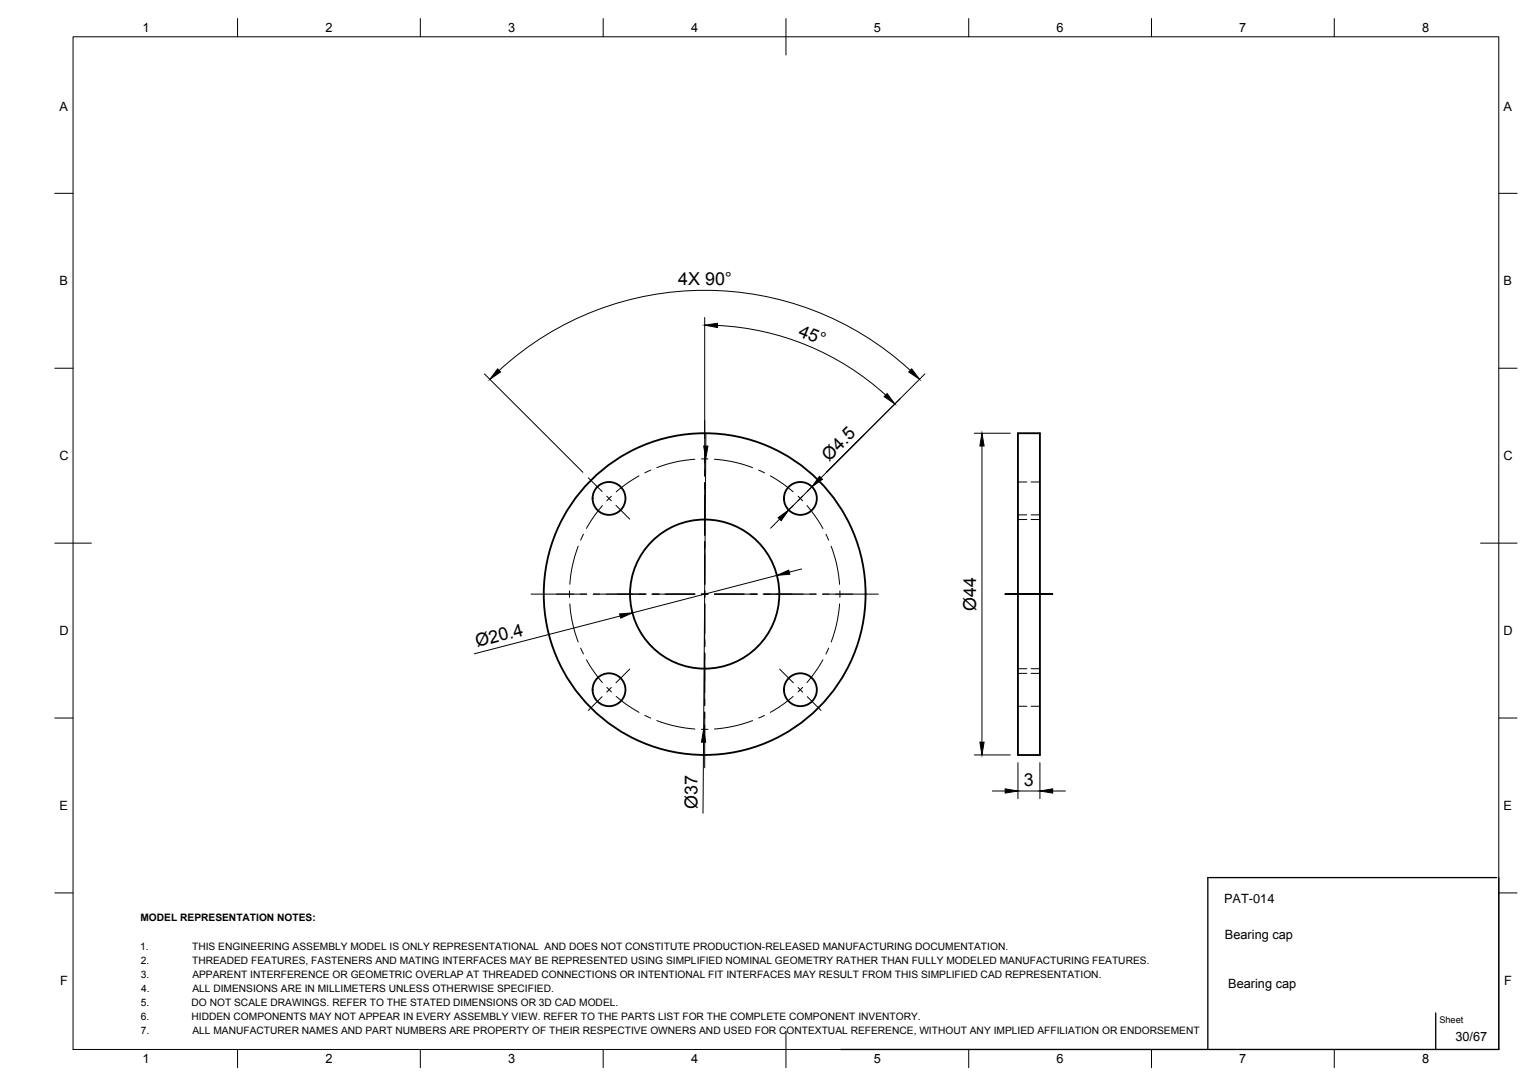
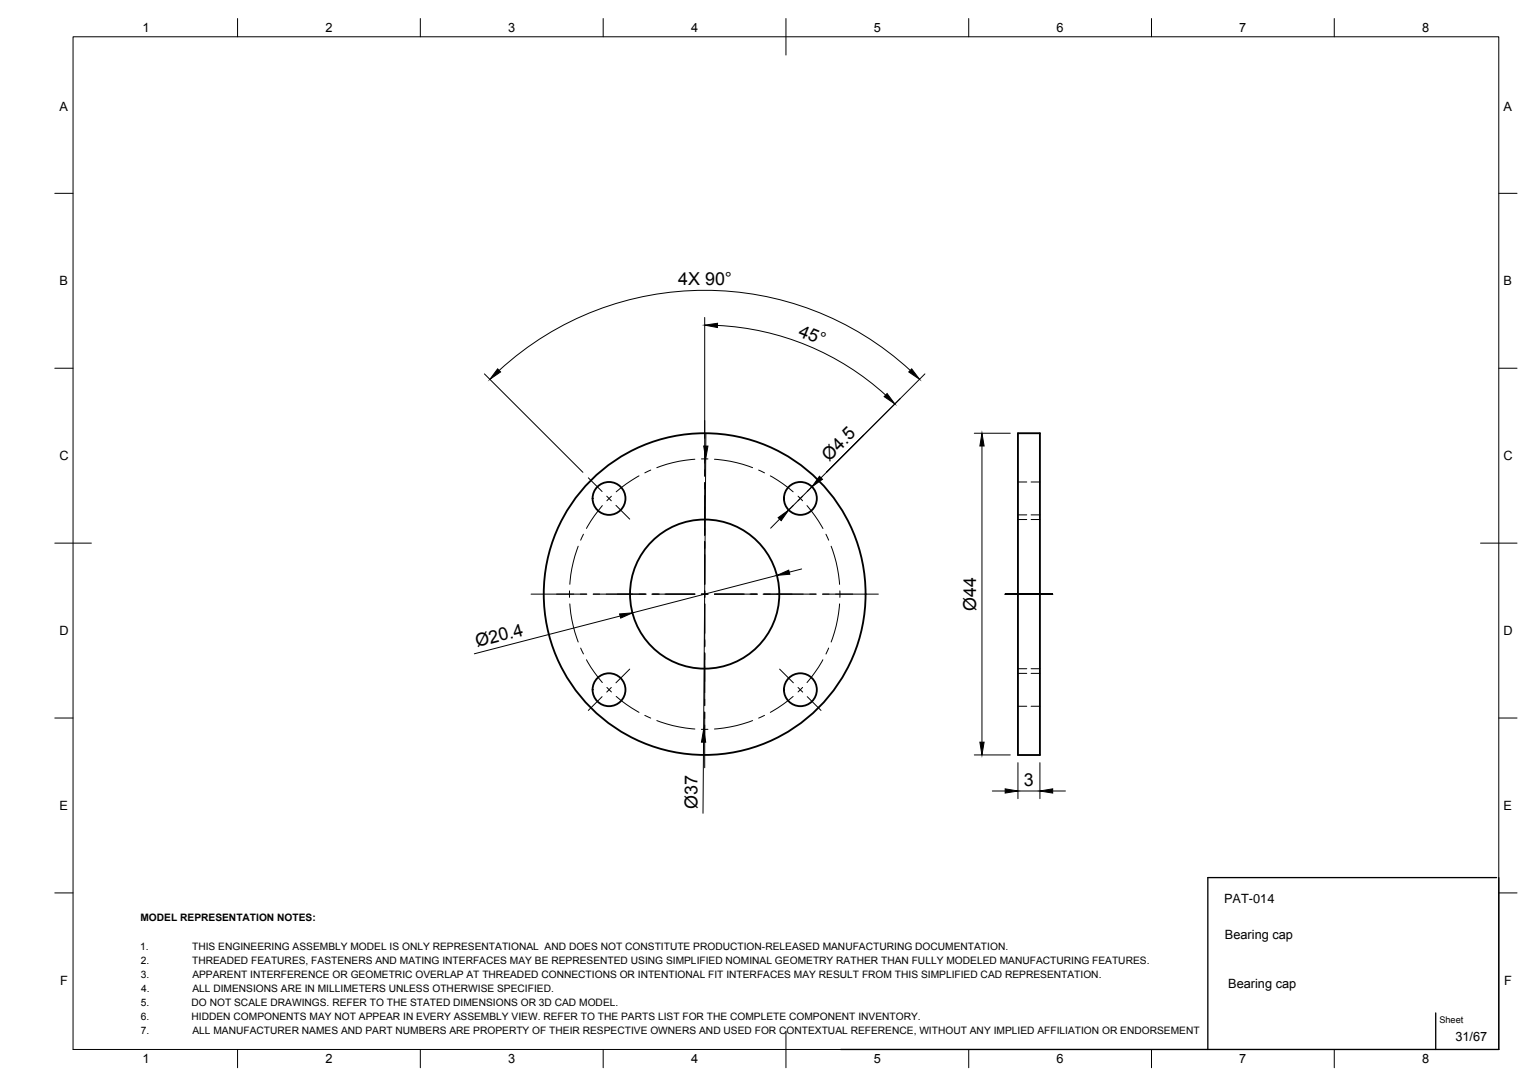
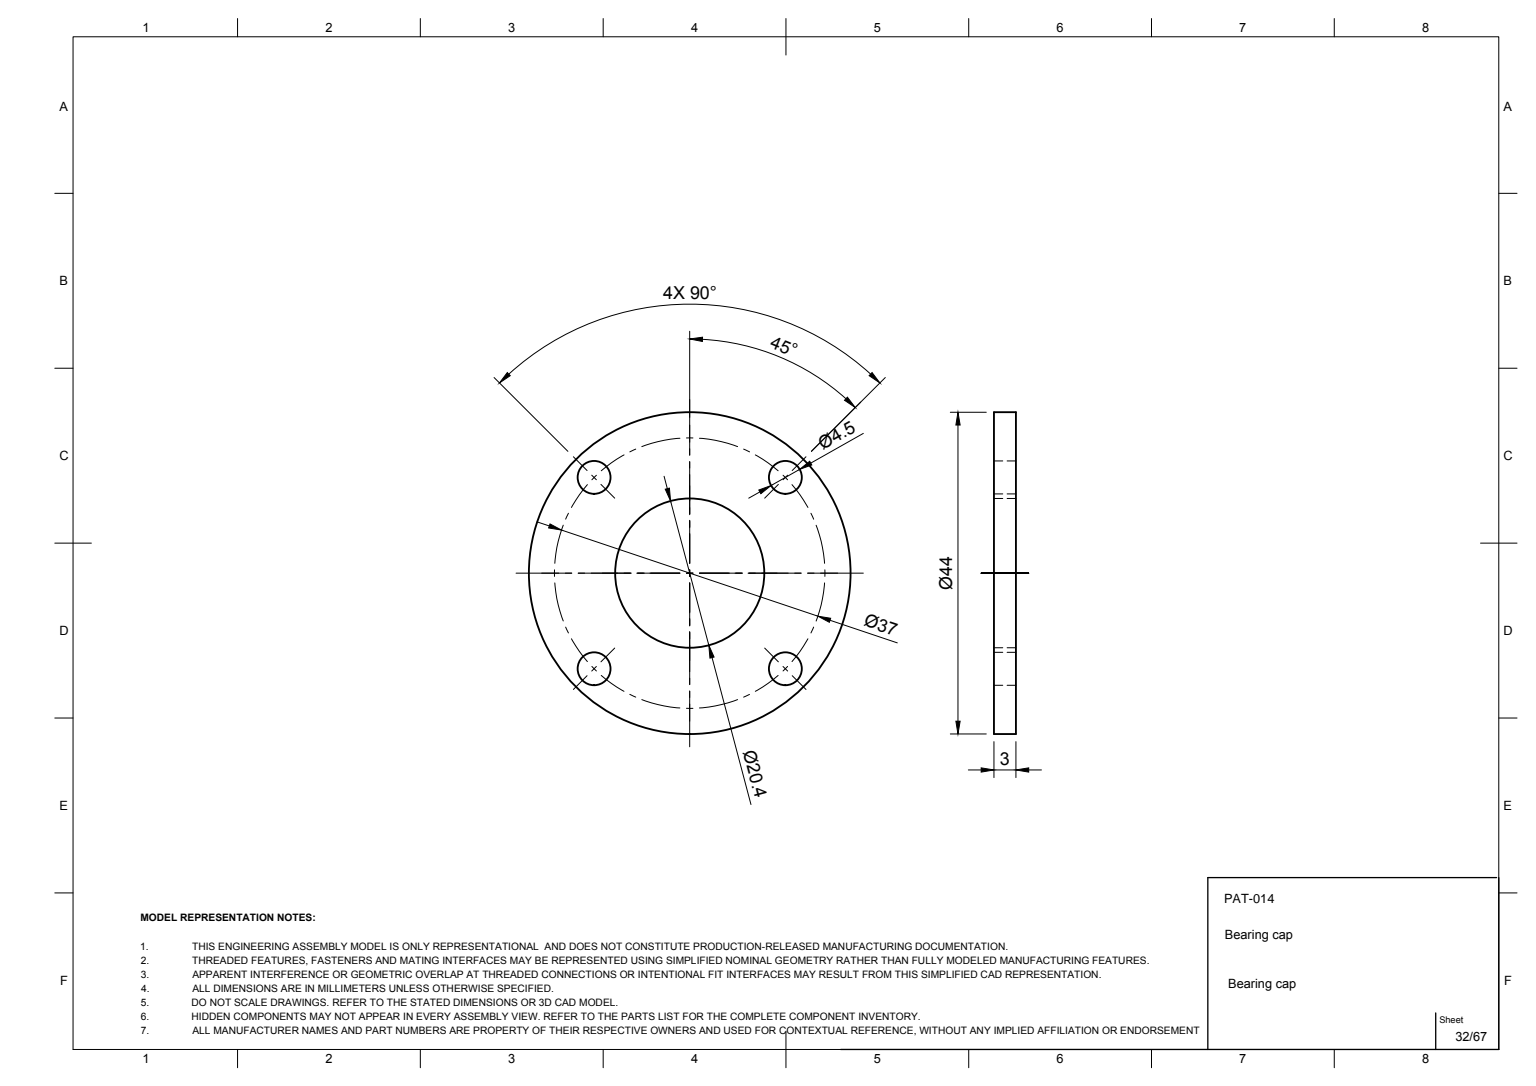
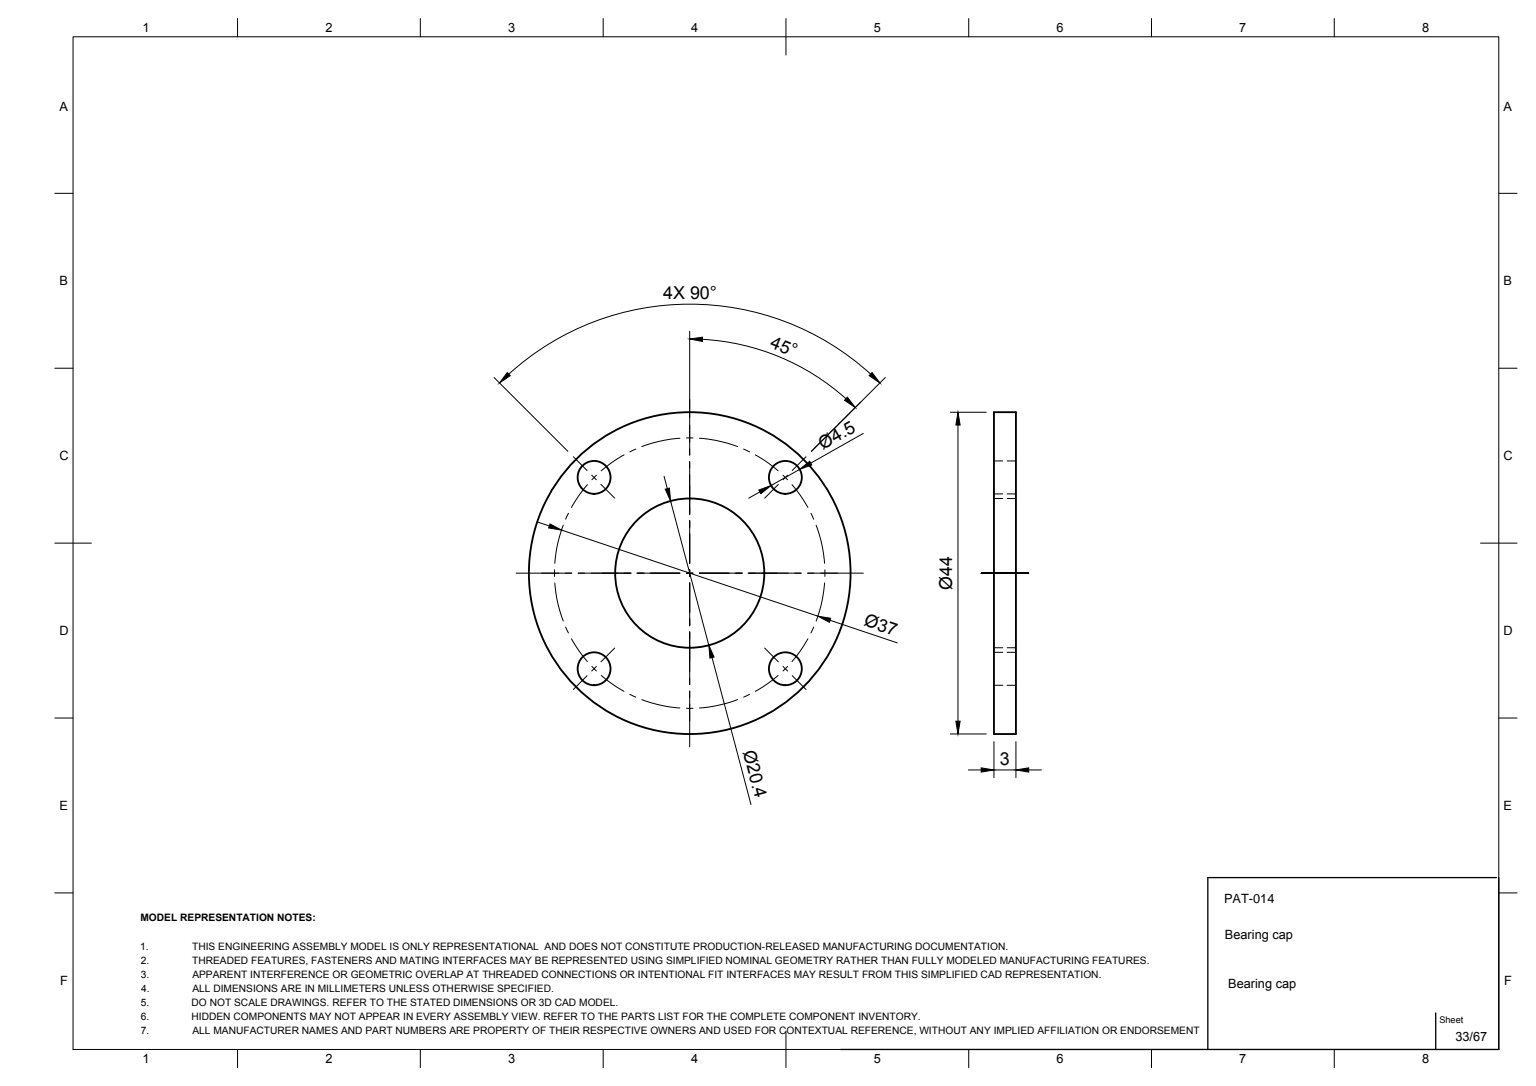
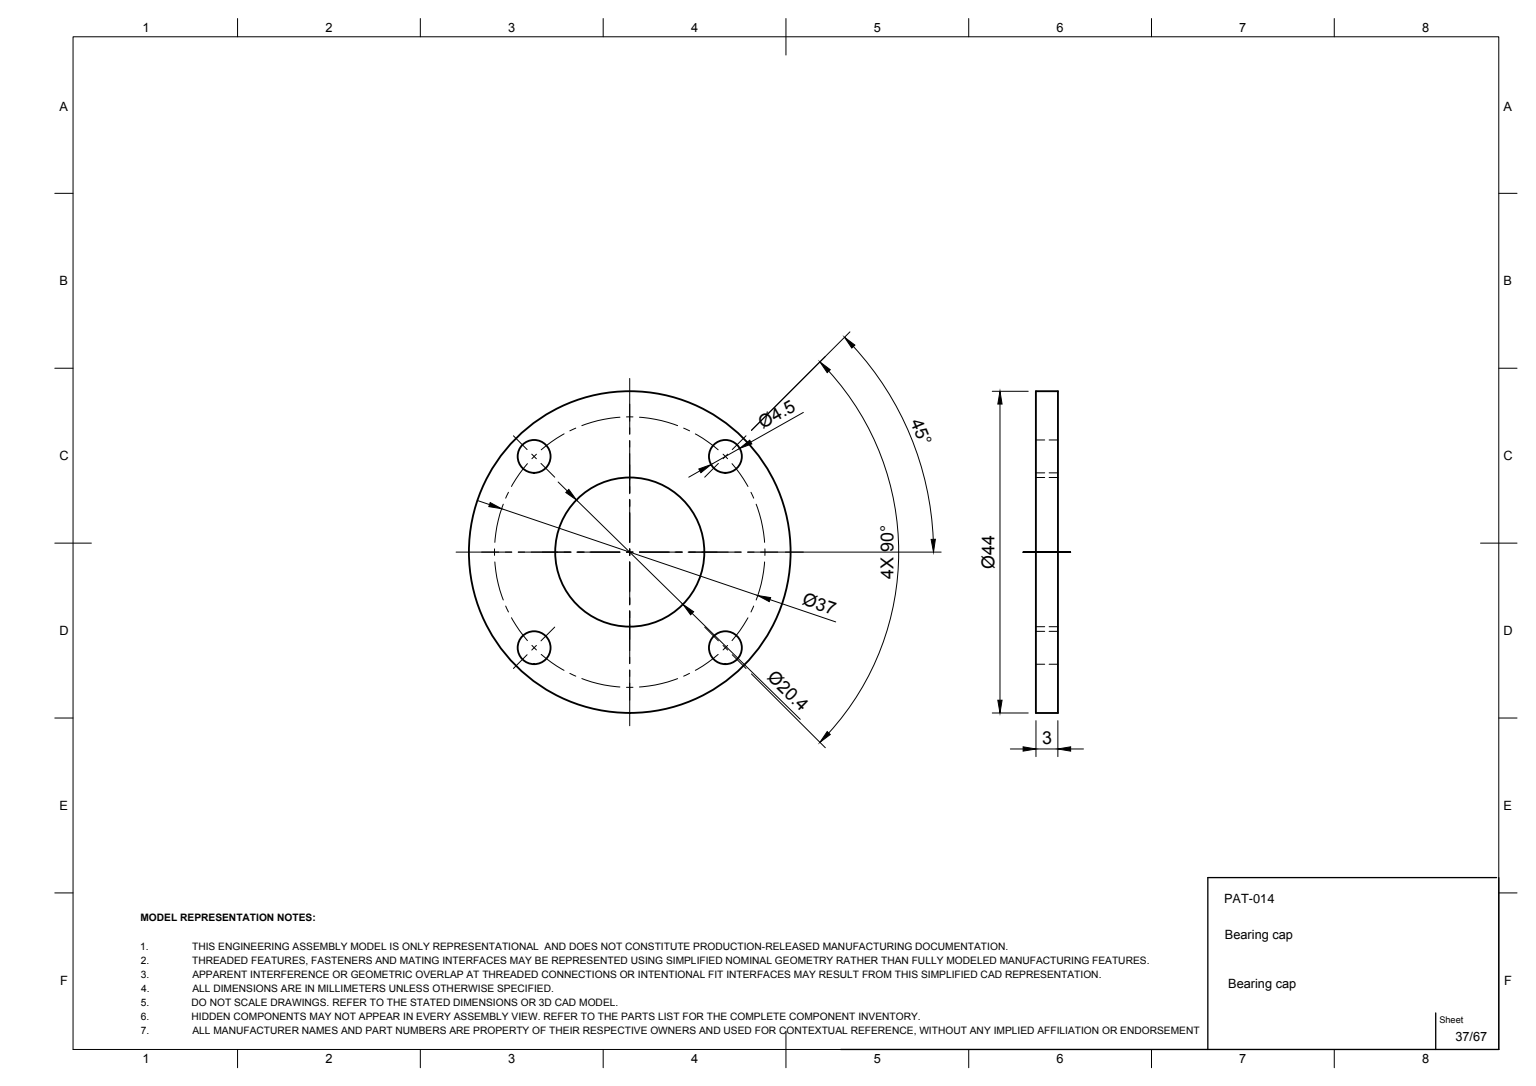
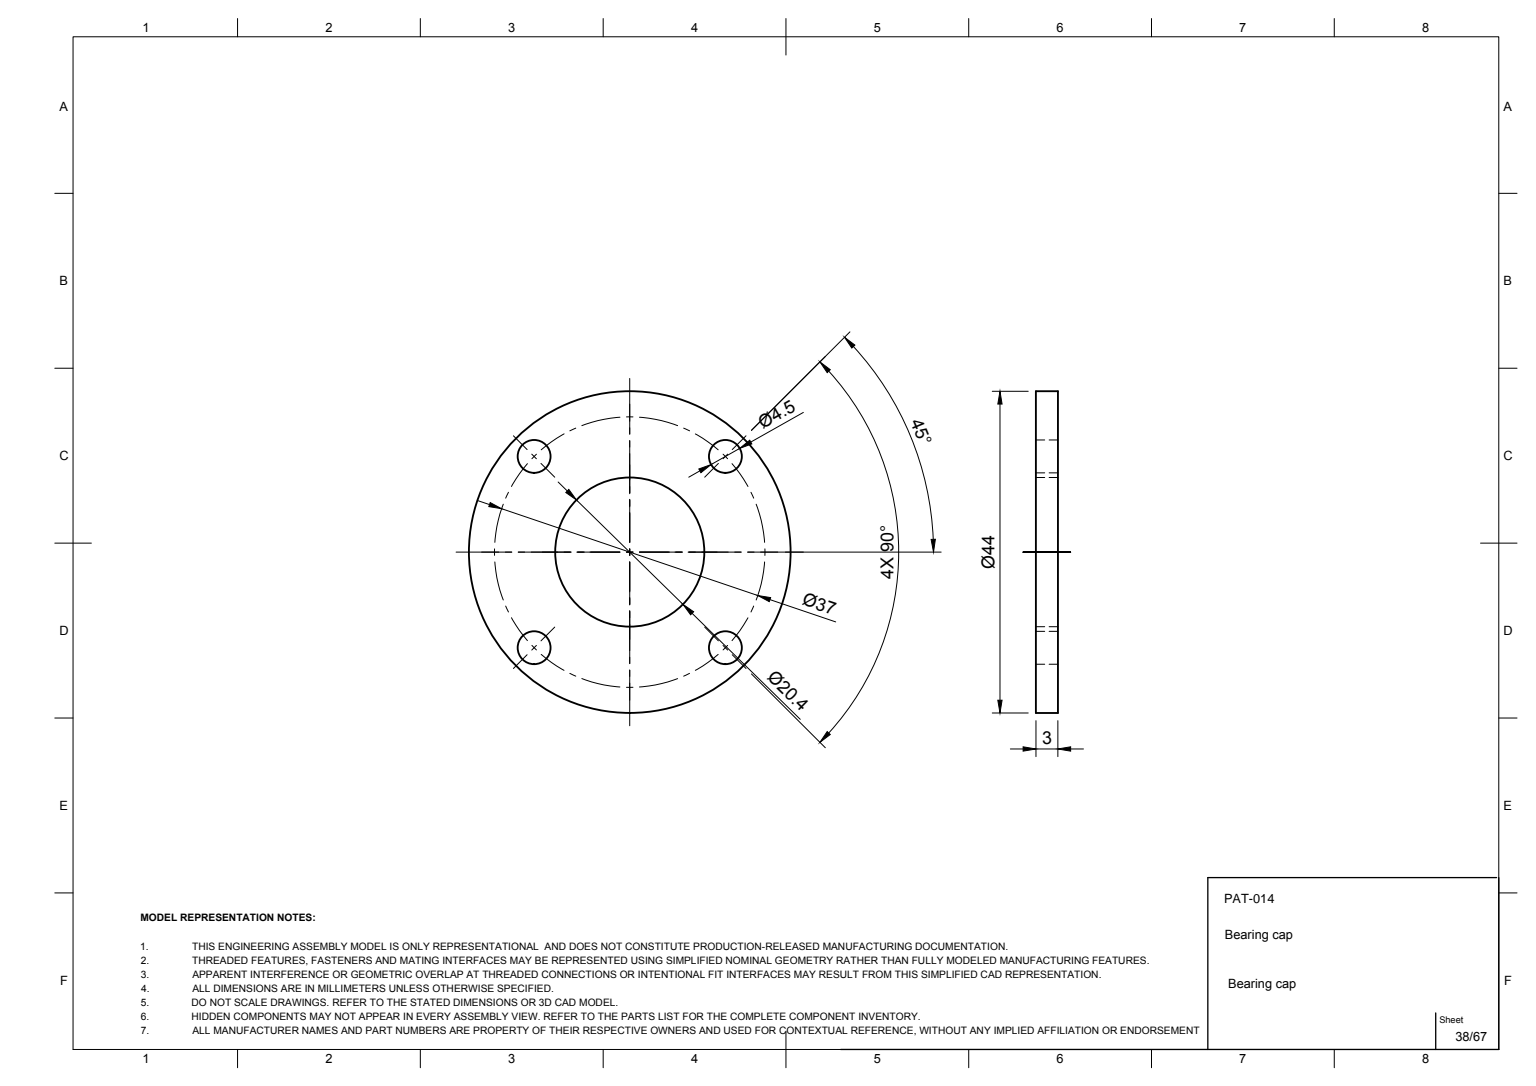
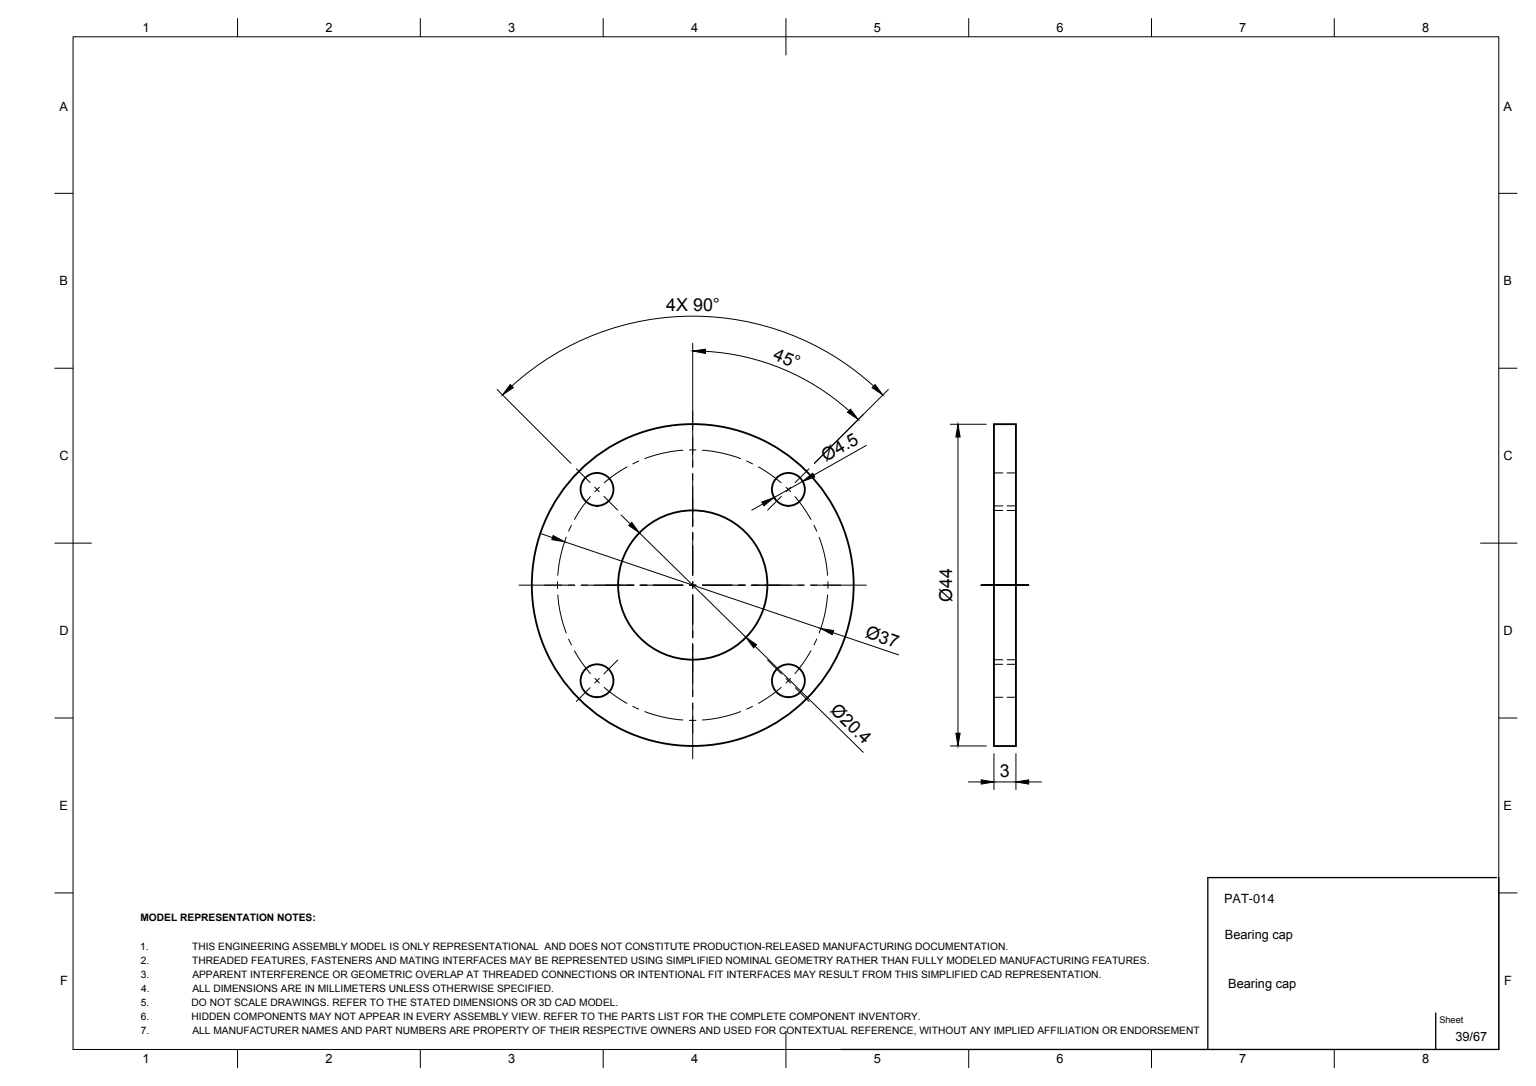
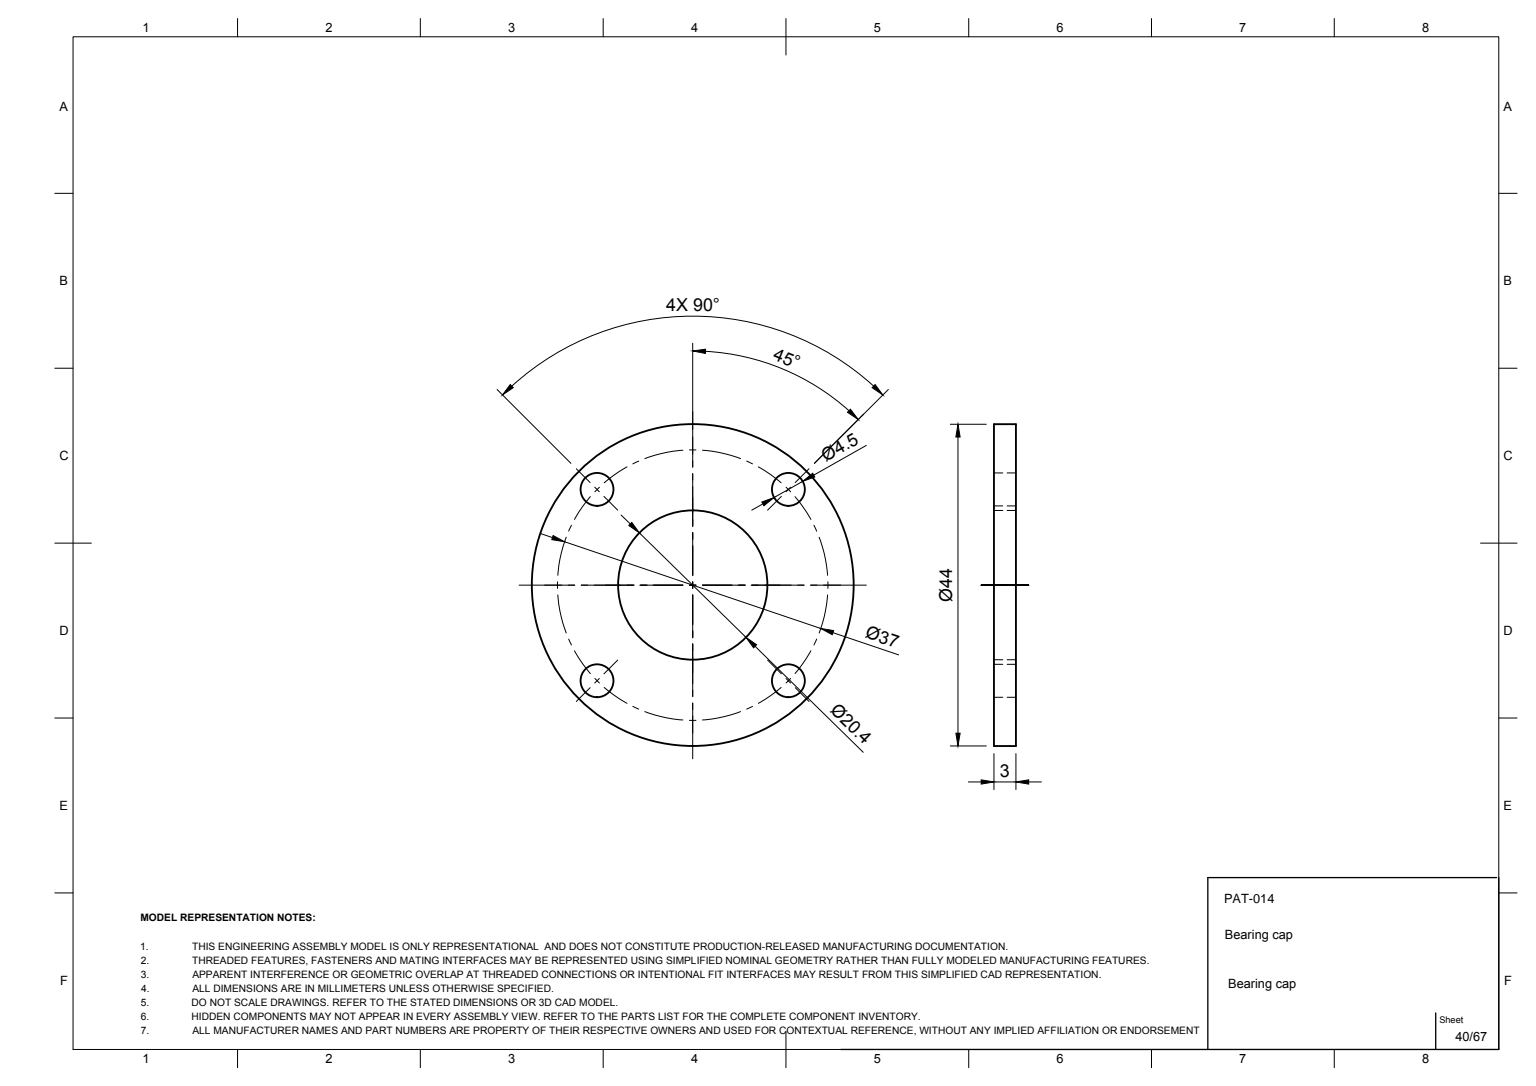
ISO-10303-21;
HEADER;
/* Generated by software containing ST-Developer
 * from STEP Tools, Inc. (www.steptools.com) 
 */

FILE_DESCRIPTION(
/* description */ ('Bin tilter linkage'),
/* implementation_level */ '2;1');

FILE_NAME(
/* name */ 'Bearing cap.step',
/* time_stamp */ '2026-10-28T03:26:24-07:00',
/* author */ (''),
/* organization */ (''),
/* preprocessor_version */ 'ST-DEVELOPER v20.2',
/* originating_system */ 'Autodesk Translation Framework v15.17.0.0',
/* authorisation */ '');

FILE_SCHEMA (('AUTOMOTIVE_DESIGN { 1 0 10303 214 3 1 1 }'));
ENDSEC;

DATA;
#10=MECHANICAL_DESIGN_GEOMETRIC_PRESENTATION_REPRESENTATION('',(#893),#23728);
#681=SHAPE_REPRESENTATION_RELATIONSHIP('SRR','None',#24146,#787);
#787=ADVANCED_BREP_SHAPE_REPRESENTATION('',(#1006),#23646);
#893=STYLED_ITEM('',(#24765),#1006);
#1006=MANIFOLD_SOLID_BREP('Body1',#12424);
#1254=FACE_BOUND('',#3106,.T.);
#1255=FACE_BOUND('',#3107,.T.);
#1256=FACE_BOUND('',#3108,.T.);
#1257=FACE_BOUND('',#3109,.T.);
#1258=FACE_BOUND('',#3110,.T.);
#1259=FACE_BOUND('',#3112,.T.);
#1260=FACE_BOUND('',#3113,.T.);
#1261=FACE_BOUND('',#3114,.T.);
#1262=FACE_BOUND('',#3115,.T.);
#1263=FACE_BOUND('',#3116,.T.);
#1621=PLANE('',#14262);
#1622=PLANE('',#14263);
#2155=FACE_OUTER_BOUND('',#3099,.T.);
#2156=FACE_OUTER_BOUND('',#3100,.T.);
#2157=FACE_OUTER_BOUND('',#3101,.T.);
#2158=FACE_OUTER_BOUND('',#3102,.T.);
#2159=FACE_OUTER_BOUND('',#3103,.T.);
#2160=FACE_OUTER_BOUND('',#3104,.T.);
#2161=FACE_OUTER_BOUND('',#3105,.T.);
#2162=FACE_OUTER_BOUND('',#3111,.T.);
#3099=EDGE_LOOP('',(#9457,#9458,#9459,#9460));
#3100=EDGE_LOOP('',(#9461,#9462,#9463,#9464));
#3101=EDGE_LOOP('',(#9465,#9466,#9467,#9468));
#3102=EDGE_LOOP('',(#9469,#9470,#9471,#9472));
#3103=EDGE_LOOP('',(#9473,#9474,#9475,#9476));
#3104=EDGE_LOOP('',(#9477,#9478,#9479,#9480));
#3105=EDGE_LOOP('',(#9481));
#3106=EDGE_LOOP('',(#9482));
#3107=EDGE_LOOP('',(#9483));
#3108=EDGE_LOOP('',(#9484));
#3109=EDGE_LOOP('',(#9485));
#3110=EDGE_LOOP('',(#9486));
#3111=EDGE_LOOP('',(#9487));
#3112=EDGE_LOOP('',(#9488));
#3113=EDGE_LOOP('',(#9489));
#3114=EDGE_LOOP('',(#9490));
#3115=EDGE_LOOP('',(#9491));
#3116=EDGE_LOOP('',(#9492));
#4123=LINE('',#20951,#4798);
#4124=LINE('',#20957,#4799);
#4125=LINE('',#20963,#4800);
#4126=LINE('',#20969,#4801);
#4127=LINE('',#20975,#4802);
#4128=LINE('',#20981,#4803);
#4798=VECTOR('',#16888,0.225);
#4799=VECTOR('',#16895,0.225);
#4800=VECTOR('',#16902,0.225);
#4801=VECTOR('',#16909,0.225);
#4802=VECTOR('',#16916,1.02);
#4803=VECTOR('',#16923,2.2);
#5467=CIRCLE('',#14245,0.225);
#5468=CIRCLE('',#14246,0.225);
#5469=CIRCLE('',#14248,0.225);
#5470=CIRCLE('',#14249,0.225);
#5471=CIRCLE('',#14251,0.225);
#5472=CIRCLE('',#14252,0.225);
#5473=CIRCLE('',#14254,0.225);
#5474=CIRCLE('',#14255,0.225);
#5475=CIRCLE('',#14257,1.02);
#5476=CIRCLE('',#14258,1.02);
#5477=CIRCLE('',#14260,2.2);
#5478=CIRCLE('',#14261,2.2);
#6317=VERTEX_POINT('',#20948);
#6318=VERTEX_POINT('',#20950);
#6319=VERTEX_POINT('',#20954);
#6320=VERTEX_POINT('',#20956);
#6321=VERTEX_POINT('',#20960);
#6322=VERTEX_POINT('',#20962);
#6323=VERTEX_POINT('',#20966);
#6324=VERTEX_POINT('',#20968);
#6325=VERTEX_POINT('',#20972);
#6326=VERTEX_POINT('',#20974);
#6327=VERTEX_POINT('',#20978);
#6328=VERTEX_POINT('',#20980);
#7468=EDGE_CURVE('',#6317,#6317,#5467,.T.);
#7469=EDGE_CURVE('',#6317,#6318,#4123,.T.);
#7470=EDGE_CURVE('',#6318,#6318,#5468,.T.);
#7471=EDGE_CURVE('',#6319,#6319,#5469,.T.);
#7472=EDGE_CURVE('',#6319,#6320,#4124,.T.);
#7473=EDGE_CURVE('',#6320,#6320,#5470,.T.);
#7474=EDGE_CURVE('',#6321,#6321,#5471,.T.);
#7475=EDGE_CURVE('',#6321,#6322,#4125,.T.);
#7476=EDGE_CURVE('',#6322,#6322,#5472,.T.);
#7477=EDGE_CURVE('',#6323,#6323,#5473,.T.);
#7478=EDGE_CURVE('',#6323,#6324,#4126,.T.);
#7479=EDGE_CURVE('',#6324,#6324,#5474,.T.);
#7480=EDGE_CURVE('',#6325,#6325,#5475,.T.);
#7481=EDGE_CURVE('',#6325,#6326,#4127,.T.);
#7482=EDGE_CURVE('',#6326,#6326,#5476,.T.);
#7483=EDGE_CURVE('',#6327,#6327,#5477,.T.);
#7484=EDGE_CURVE('',#6327,#6328,#4128,.T.);
#7485=EDGE_CURVE('',#6328,#6328,#5478,.T.);
#9457=ORIENTED_EDGE('',*,*,#7468,.F.);
#9458=ORIENTED_EDGE('',*,*,#7469,.T.);
#9459=ORIENTED_EDGE('',*,*,#7470,.F.);
#9460=ORIENTED_EDGE('',*,*,#7469,.F.);
#9461=ORIENTED_EDGE('',*,*,#7471,.F.);
#9462=ORIENTED_EDGE('',*,*,#7472,.T.);
#9463=ORIENTED_EDGE('',*,*,#7473,.F.);
#9464=ORIENTED_EDGE('',*,*,#7472,.F.);
#9465=ORIENTED_EDGE('',*,*,#7474,.F.);
#9466=ORIENTED_EDGE('',*,*,#7475,.T.);
#9467=ORIENTED_EDGE('',*,*,#7476,.F.);
#9468=ORIENTED_EDGE('',*,*,#7475,.F.);
#9469=ORIENTED_EDGE('',*,*,#7477,.F.);
#9470=ORIENTED_EDGE('',*,*,#7478,.T.);
#9471=ORIENTED_EDGE('',*,*,#7479,.F.);
#9472=ORIENTED_EDGE('',*,*,#7478,.F.);
#9473=ORIENTED_EDGE('',*,*,#7480,.F.);
#9474=ORIENTED_EDGE('',*,*,#7481,.T.);
#9475=ORIENTED_EDGE('',*,*,#7482,.T.);
#9476=ORIENTED_EDGE('',*,*,#7481,.F.);
#9477=ORIENTED_EDGE('',*,*,#7483,.F.);
#9478=ORIENTED_EDGE('',*,*,#7484,.T.);
#9479=ORIENTED_EDGE('',*,*,#7485,.T.);
#9480=ORIENTED_EDGE('',*,*,#7484,.F.);
#9481=ORIENTED_EDGE('',*,*,#7483,.T.);
#9482=ORIENTED_EDGE('',*,*,#7480,.T.);
#9483=ORIENTED_EDGE('',*,*,#7479,.T.);
#9484=ORIENTED_EDGE('',*,*,#7476,.T.);
#9485=ORIENTED_EDGE('',*,*,#7473,.T.);
#9486=ORIENTED_EDGE('',*,*,#7470,.T.);
#9487=ORIENTED_EDGE('',*,*,#7485,.F.);
#9488=ORIENTED_EDGE('',*,*,#7482,.F.);
#9489=ORIENTED_EDGE('',*,*,#7477,.T.);
#9490=ORIENTED_EDGE('',*,*,#7474,.T.);
#9491=ORIENTED_EDGE('',*,*,#7471,.T.);
#9492=ORIENTED_EDGE('',*,*,#7468,.T.);
#11399=CYLINDRICAL_SURFACE('',#14244,0.225);
#11400=CYLINDRICAL_SURFACE('',#14247,0.225);
#11401=CYLINDRICAL_SURFACE('',#14250,0.225);
#11402=CYLINDRICAL_SURFACE('',#14253,0.225);
#11403=CYLINDRICAL_SURFACE('',#14256,1.02);
#11404=CYLINDRICAL_SURFACE('',#14259,2.2);
#11880=ADVANCED_FACE('',(#2155),#11399,.F.);
#11881=ADVANCED_FACE('',(#2156),#11400,.F.);
#11882=ADVANCED_FACE('',(#2157),#11401,.F.);
#11883=ADVANCED_FACE('',(#2158),#11402,.F.);
#11884=ADVANCED_FACE('',(#2159),#11403,.F.);
#11885=ADVANCED_FACE('',(#2160),#11404,.T.);
#11886=ADVANCED_FACE('',(#2161,#1254,#1255,#1256,#1257,#1258),#1621,.T.);
#11887=ADVANCED_FACE('',(#2162,#1259,#1260,#1261,#1262,#1263),#1622,.F.);
#12424=CLOSED_SHELL('',(#11880,#11881,#11882,#11883,#11884,#11885,#11886,
#11887));
#14243=AXIS2_PLACEMENT_3D('',#20946,#16882,#16883);
#14244=AXIS2_PLACEMENT_3D('',#20947,#16884,#16885);
#14245=AXIS2_PLACEMENT_3D('',#20949,#16886,#16887);
#14246=AXIS2_PLACEMENT_3D('',#20952,#16889,#16890);
#14247=AXIS2_PLACEMENT_3D('',#20953,#16891,#16892);
#14248=AXIS2_PLACEMENT_3D('',#20955,#16893,#16894);
#14249=AXIS2_PLACEMENT_3D('',#20958,#16896,#16897);
#14250=AXIS2_PLACEMENT_3D('',#20959,#16898,#16899);
#14251=AXIS2_PLACEMENT_3D('',#20961,#16900,#16901);
#14252=AXIS2_PLACEMENT_3D('',#20964,#16903,#16904);
#14253=AXIS2_PLACEMENT_3D('',#20965,#16905,#16906);
#14254=AXIS2_PLACEMENT_3D('',#20967,#16907,#16908);
#14255=AXIS2_PLACEMENT_3D('',#20970,#16910,#16911);
#14256=AXIS2_PLACEMENT_3D('',#20971,#16912,#16913);
#14257=AXIS2_PLACEMENT_3D('',#20973,#16914,#16915);
#14258=AXIS2_PLACEMENT_3D('',#20976,#16917,#16918);
#14259=AXIS2_PLACEMENT_3D('',#20977,#16919,#16920);
#14260=AXIS2_PLACEMENT_3D('',#20979,#16921,#16922);
#14261=AXIS2_PLACEMENT_3D('',#20982,#16924,#16925);
#14262=AXIS2_PLACEMENT_3D('',#20983,#16926,#16927);
#14263=AXIS2_PLACEMENT_3D('',#20984,#16928,#16929);
#16882=DIRECTION('axis',(0.,0.,1.));
#16883=DIRECTION('refdir',(1.,0.,0.));
#16884=DIRECTION('center_axis',(0.,1.,0.));
#16885=DIRECTION('ref_axis',(1.,0.,0.));
#16886=DIRECTION('center_axis',(0.,1.,0.));
#16887=DIRECTION('ref_axis',(1.,0.,0.));
#16888=DIRECTION('',(0.,1.,0.));
#16889=DIRECTION('center_axis',(0.,-1.,0.));
#16890=DIRECTION('ref_axis',(1.,0.,0.));
#16891=DIRECTION('center_axis',(0.,1.,0.));
#16892=DIRECTION('ref_axis',(1.,0.,0.));
#16893=DIRECTION('center_axis',(0.,1.,0.));
#16894=DIRECTION('ref_axis',(1.,0.,0.));
#16895=DIRECTION('',(0.,1.,0.));
#16896=DIRECTION('center_axis',(0.,-1.,0.));
#16897=DIRECTION('ref_axis',(1.,0.,0.));
#16898=DIRECTION('center_axis',(0.,1.,0.));
#16899=DIRECTION('ref_axis',(1.,0.,0.));
#16900=DIRECTION('center_axis',(0.,1.,0.));
#16901=DIRECTION('ref_axis',(1.,0.,0.));
#16902=DIRECTION('',(0.,1.,0.));
#16903=DIRECTION('center_axis',(0.,-1.,0.));
#16904=DIRECTION('ref_axis',(1.,0.,0.));
#16905=DIRECTION('center_axis',(0.,1.,0.));
#16906=DIRECTION('ref_axis',(1.,0.,0.));
#16907=DIRECTION('center_axis',(0.,1.,0.));
#16908=DIRECTION('ref_axis',(1.,0.,0.));
#16909=DIRECTION('',(0.,1.,0.));
#16910=DIRECTION('center_axis',(0.,-1.,0.));
#16911=DIRECTION('ref_axis',(1.,0.,0.));
#16912=DIRECTION('center_axis',(0.,1.,0.));
#16913=DIRECTION('ref_axis',(1.,0.,0.));
#16914=DIRECTION('center_axis',(0.,-1.,0.));
#16915=DIRECTION('ref_axis',(1.,0.,0.));
#16916=DIRECTION('',(0.,-1.,0.));
#16917=DIRECTION('center_axis',(0.,-1.,0.));
#16918=DIRECTION('ref_axis',(1.,0.,0.));
#16919=DIRECTION('center_axis',(0.,1.,0.));
#16920=DIRECTION('ref_axis',(1.,0.,0.));
#16921=DIRECTION('center_axis',(0.,1.,0.));
#16922=DIRECTION('ref_axis',(1.,0.,0.));
#16923=DIRECTION('',(0.,-1.,0.));
#16924=DIRECTION('center_axis',(0.,1.,0.));
#16925=DIRECTION('ref_axis',(1.,0.,0.));
#16926=DIRECTION('center_axis',(0.,1.,0.));
#16927=DIRECTION('ref_axis',(1.,0.,0.));
#16928=DIRECTION('center_axis',(0.,1.,0.));
#16929=DIRECTION('ref_axis',(1.,0.,0.));
#20946=CARTESIAN_POINT('',(0.,0.,0.));
#20947=CARTESIAN_POINT('Origin',(-1.30814754519511,-0.9,13.6918524548049));
#20948=CARTESIAN_POINT('',(-1.53314754519511,-0.8,13.6918524548049));
#20949=CARTESIAN_POINT('Origin',(-1.30814754519511,-0.8,13.6918524548049));
#20950=CARTESIAN_POINT('',(-1.53314754519511,-0.5,13.6918524548049));
#20951=CARTESIAN_POINT('',(-1.53314754519511,-0.9,13.6918524548049));
#20952=CARTESIAN_POINT('Origin',(-1.30814754519511,-0.5,13.6918524548049));
#20953=CARTESIAN_POINT('Origin',(-1.30814754519511,-0.9,16.3081475451951));
#20954=CARTESIAN_POINT('',(-1.53314754519511,-0.8,16.3081475451951));
#20955=CARTESIAN_POINT('Origin',(-1.30814754519511,-0.8,16.3081475451951));
#20956=CARTESIAN_POINT('',(-1.53314754519511,-0.5,16.3081475451951));
#20957=CARTESIAN_POINT('',(-1.53314754519511,-0.9,16.3081475451951));
#20958=CARTESIAN_POINT('Origin',(-1.30814754519511,-0.5,16.3081475451951));
#20959=CARTESIAN_POINT('Origin',(1.30814754519511,-0.9,16.3081475451951));
#20960=CARTESIAN_POINT('',(1.08314754519511,-0.8,16.3081475451951));
#20961=CARTESIAN_POINT('Origin',(1.30814754519511,-0.8,16.3081475451951));
#20962=CARTESIAN_POINT('',(1.08314754519511,-0.5,16.3081475451951));
#20963=CARTESIAN_POINT('',(1.08314754519511,-0.9,16.3081475451951));
#20964=CARTESIAN_POINT('Origin',(1.30814754519511,-0.5,16.3081475451951));
#20965=CARTESIAN_POINT('Origin',(1.30814754519511,-0.9,13.6918524548049));
#20966=CARTESIAN_POINT('',(1.08314754519511,-0.8,13.6918524548049));
#20967=CARTESIAN_POINT('Origin',(1.30814754519511,-0.8,13.6918524548049));
#20968=CARTESIAN_POINT('',(1.08314754519511,-0.5,13.6918524548049));
#20969=CARTESIAN_POINT('',(1.08314754519511,-0.9,13.6918524548049));
#20970=CARTESIAN_POINT('Origin',(1.30814754519511,-0.5,13.6918524548049));
#20971=CARTESIAN_POINT('Origin',(0.,-0.8,15.));
#20972=CARTESIAN_POINT('',(-1.02,-0.5,15.));
#20973=CARTESIAN_POINT('Origin',(0.,-0.5,15.));
#20974=CARTESIAN_POINT('',(-1.02,-0.8,15.));
#20975=CARTESIAN_POINT('',(-1.02,-0.8,15.));
#20976=CARTESIAN_POINT('Origin',(0.,-0.8,15.));
#20977=CARTESIAN_POINT('Origin',(0.,-0.8,15.));
#20978=CARTESIAN_POINT('',(-2.2,-0.5,15.));
#20979=CARTESIAN_POINT('Origin',(0.,-0.5,15.));
#20980=CARTESIAN_POINT('',(-2.2,-0.8,15.));
#20981=CARTESIAN_POINT('',(-2.2,-0.8,15.));
#20982=CARTESIAN_POINT('Origin',(0.,-0.8,15.));
#20983=CARTESIAN_POINT('Origin',(0.,-0.5,15.));
#20984=CARTESIAN_POINT('Origin',(0.,-0.8,15.));
#23529=UNCERTAINTY_MEASURE_WITH_UNIT(LENGTH_MEASURE(0.001),#23729,
'DISTANCE_ACCURACY_VALUE',
'Maximum model space distance between geometric entities at asserted c
onnectivities');
#23611=UNCERTAINTY_MEASURE_WITH_UNIT(LENGTH_MEASURE(0.001),#23729,
'DISTANCE_ACCURACY_VALUE',
'Maximum model space distance between geometric entities at asserted c
onnectivities');
#23646=(
GEOMETRIC_REPRESENTATION_CONTEXT(3)
GLOBAL_UNCERTAINTY_ASSIGNED_CONTEXT((#23529))
GLOBAL_UNIT_ASSIGNED_CONTEXT((#23729,#23731,#23732))
REPRESENTATION_CONTEXT('','3D')
);
#23728=(
GEOMETRIC_REPRESENTATION_CONTEXT(3)
GLOBAL_UNCERTAINTY_ASSIGNED_CONTEXT((#23611))
GLOBAL_UNIT_ASSIGNED_CONTEXT((#23729,#23731,#23732))
REPRESENTATION_CONTEXT('','3D')
);
#23729=(
LENGTH_UNIT()
NAMED_UNIT(*)
SI_UNIT(.CENTI.,.METRE.)
);
#23731=(
NAMED_UNIT(*)
PLANE_ANGLE_UNIT()
SI_UNIT($,.RADIAN.)
);
#23732=(
NAMED_UNIT(*)
SI_UNIT($,.STERADIAN.)
SOLID_ANGLE_UNIT()
);
#23767=SHAPE_DEFINITION_REPRESENTATION(#23883,#24146);
#23883=PRODUCT_DEFINITION_SHAPE('',$,#24263);
#24146=SHAPE_REPRESENTATION('',(#14243),#23646);
#24228=PRODUCT_DEFINITION_CONTEXT('part definition',#24578,'design');
#24263=PRODUCT_DEFINITION('Bearing cap','Bearing cap',#24379,#24228);
#24379=PRODUCT_DEFINITION_FORMATION('',$,#24614);
#24578=APPLICATION_CONTEXT(
'Core Data for Automotive Mechanical Design Process');
#24579=PRODUCT_CONTEXT('part definition',#24578,'mechanical');
#24614=PRODUCT('Bearing cap','Bearing cap','Bearing cap',(#24579));
#24759=COLOUR_RGB('Grey',0.48,0.52,0.57);
#24760=FILL_AREA_STYLE_COLOUR('',#24759);
#24761=FILL_AREA_STYLE('',(#24760));
#24762=SURFACE_STYLE_FILL_AREA(#24761);
#24763=SURFACE_SIDE_STYLE('',(#24762));
#24764=SURFACE_STYLE_USAGE(.BOTH.,#24763);
#24765=PRESENTATION_STYLE_ASSIGNMENT((#24764));
ENDSEC;
END-ISO-10303-21;
